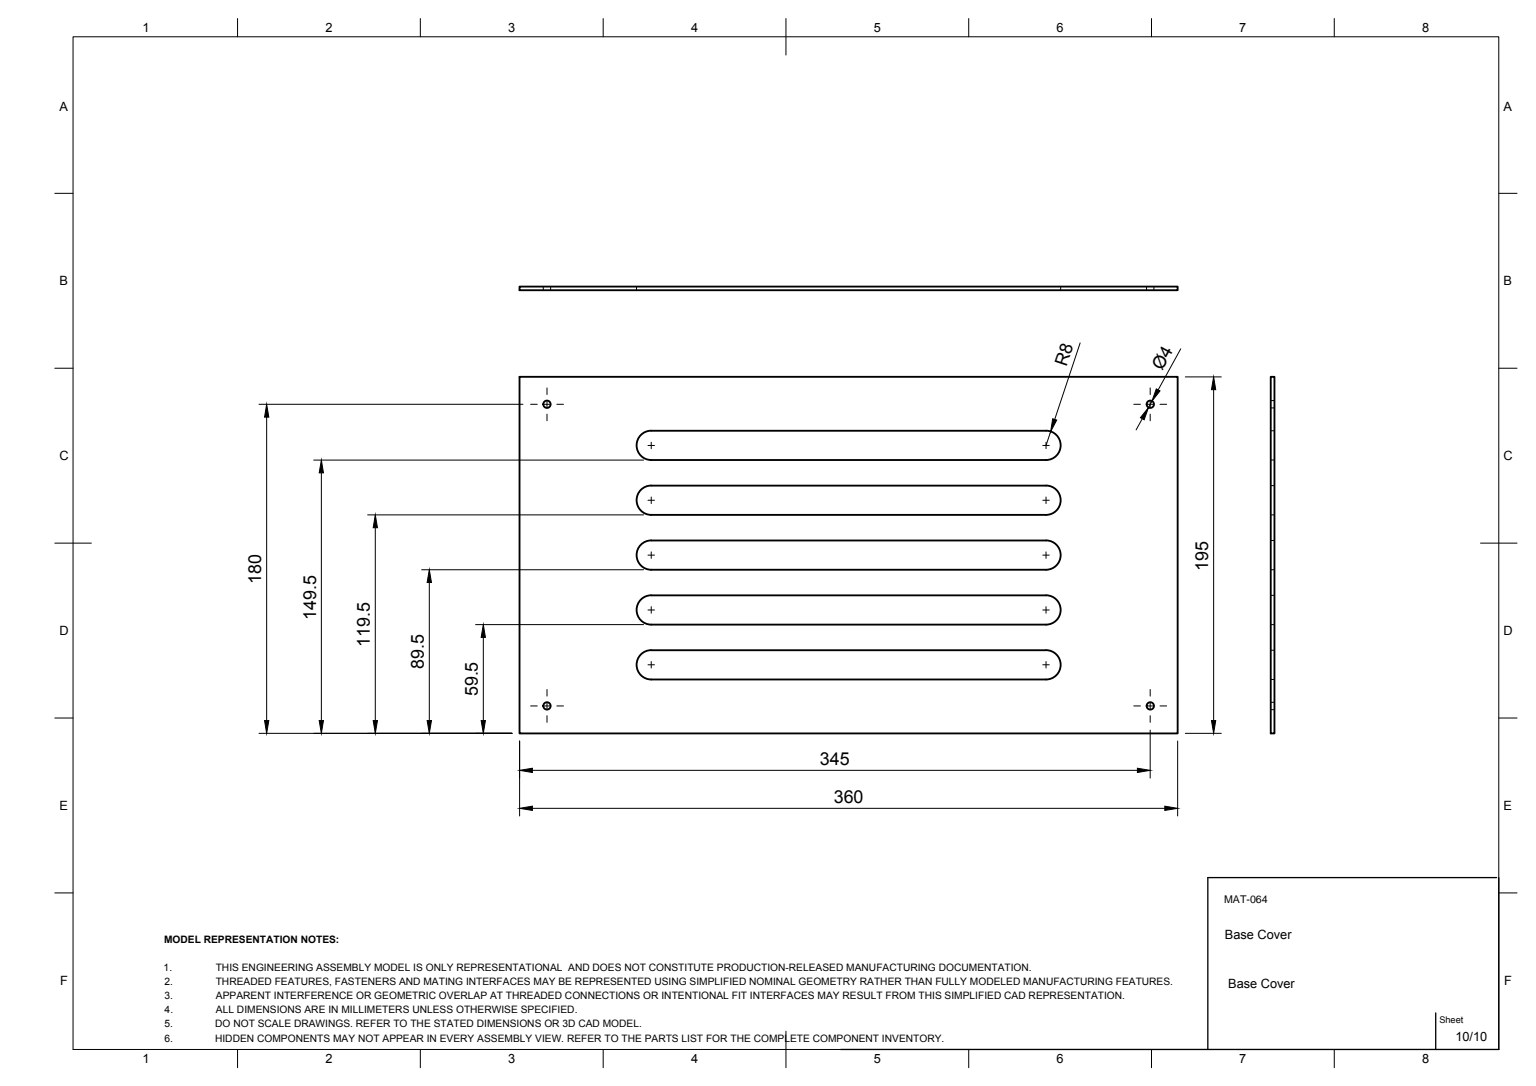
ISO-10303-21;
HEADER;
/* Generated by software containing ST-Developer
 * from STEP Tools, Inc. (www.steptools.com) 
 */

FILE_DESCRIPTION(
/* description */ (''),
/* implementation_level */ '2;1');

FILE_NAME(
/* name */ 
'Base Cover.step',
/* time_stamp */ '2026-10-24T12:42:14-07:00',
/* author */ (''),
/* organization */ (''),
/* preprocessor_version */ 'ST-DEVELOPER v20.2',
/* originating_system */ 'Autodesk Translation Framework v15.15.0.0',
/* authorisation */ '');

FILE_SCHEMA (('AUTOMOTIVE_DESIGN { 1 0 10303 214 3 1 1 }'));
ENDSEC;

DATA;
#10=MECHANICAL_DESIGN_GEOMETRIC_PRESENTATION_REPRESENTATION('',(#67),#6789);
#55=SHAPE_REPRESENTATION_RELATIONSHIP('SRR','None',#6822,#61);
#61=ADVANCED_BREP_SHAPE_REPRESENTATION('',(#73),#6784);
#67=STYLED_ITEM('',(#6863),#73);
#73=MANIFOLD_SOLID_BREP('Base Cover',#3962);
#146=CYLINDRICAL_SURFACE('',#4260,2.);
#147=CYLINDRICAL_SURFACE('',#4261,2.);
#148=CYLINDRICAL_SURFACE('',#4262,2.);
#149=CYLINDRICAL_SURFACE('',#4263,2.);
#150=CYLINDRICAL_SURFACE('',#4264,7.99999999999998);
#151=CYLINDRICAL_SURFACE('',#4266,8.00000000000009);
#152=CYLINDRICAL_SURFACE('',#4268,8.00000000000009);
#153=CYLINDRICAL_SURFACE('',#4270,8.00000000000004);
#154=CYLINDRICAL_SURFACE('',#4272,7.99999999999998);
#155=CYLINDRICAL_SURFACE('',#4274,8.00000000000009);
#156=CYLINDRICAL_SURFACE('',#4276,8.00000000000009);
#157=CYLINDRICAL_SURFACE('',#4278,8.00000000000004);
#158=CYLINDRICAL_SURFACE('',#4280,8.00000000000004);
#159=CYLINDRICAL_SURFACE('',#4282,8.00000000000004);
#201=FACE_BOUND('',#752,.T.);
#202=FACE_BOUND('',#753,.T.);
#203=FACE_BOUND('',#754,.T.);
#204=FACE_BOUND('',#755,.T.);
#205=FACE_BOUND('',#756,.T.);
#206=FACE_BOUND('',#757,.T.);
#207=FACE_BOUND('',#758,.T.);
#208=FACE_BOUND('',#759,.T.);
#209=FACE_BOUND('',#760,.T.);
#210=FACE_BOUND('',#762,.T.);
#211=FACE_BOUND('',#763,.T.);
#212=FACE_BOUND('',#764,.T.);
#213=FACE_BOUND('',#765,.T.);
#214=FACE_BOUND('',#766,.T.);
#215=FACE_BOUND('',#767,.T.);
#216=FACE_BOUND('',#768,.T.);
#217=FACE_BOUND('',#769,.T.);
#218=FACE_BOUND('',#770,.T.);
#294=CIRCLE('',#4231,8.00000000000004);
#295=CIRCLE('',#4232,8.00000000000004);
#296=CIRCLE('',#4233,8.00000000000009);
#297=CIRCLE('',#4234,8.00000000000004);
#298=CIRCLE('',#4235,7.99999999999998);
#299=CIRCLE('',#4236,8.00000000000009);
#300=CIRCLE('',#4237,8.00000000000009);
#301=CIRCLE('',#4238,8.00000000000004);
#302=CIRCLE('',#4239,7.99999999999998);
#303=CIRCLE('',#4240,8.00000000000009);
#304=CIRCLE('',#4241,2.);
#305=CIRCLE('',#4242,2.);
#306=CIRCLE('',#4243,2.);
#307=CIRCLE('',#4244,2.);
#308=CIRCLE('',#4246,8.00000000000004);
#309=CIRCLE('',#4247,8.00000000000004);
#310=CIRCLE('',#4248,8.00000000000009);
#311=CIRCLE('',#4249,8.00000000000004);
#312=CIRCLE('',#4250,7.99999999999998);
#313=CIRCLE('',#4251,8.00000000000009);
#314=CIRCLE('',#4252,8.00000000000009);
#315=CIRCLE('',#4253,8.00000000000004);
#316=CIRCLE('',#4254,7.99999999999998);
#317=CIRCLE('',#4255,8.00000000000009);
#318=CIRCLE('',#4256,2.);
#319=CIRCLE('',#4257,2.);
#320=CIRCLE('',#4258,2.);
#321=CIRCLE('',#4259,2.);
#514=FACE_OUTER_BOUND('',#747,.T.);
#515=FACE_OUTER_BOUND('',#748,.T.);
#516=FACE_OUTER_BOUND('',#749,.T.);
#517=FACE_OUTER_BOUND('',#750,.T.);
#518=FACE_OUTER_BOUND('',#751,.T.);
#519=FACE_OUTER_BOUND('',#761,.T.);
#520=FACE_OUTER_BOUND('',#771,.T.);
#521=FACE_OUTER_BOUND('',#772,.T.);
#522=FACE_OUTER_BOUND('',#773,.T.);
#523=FACE_OUTER_BOUND('',#774,.T.);
#524=FACE_OUTER_BOUND('',#775,.T.);
#525=FACE_OUTER_BOUND('',#776,.T.);
#526=FACE_OUTER_BOUND('',#777,.T.);
#527=FACE_OUTER_BOUND('',#778,.T.);
#528=FACE_OUTER_BOUND('',#779,.T.);
#529=FACE_OUTER_BOUND('',#780,.T.);
#530=FACE_OUTER_BOUND('',#781,.T.);
#531=FACE_OUTER_BOUND('',#782,.T.);
#532=FACE_OUTER_BOUND('',#783,.T.);
#533=FACE_OUTER_BOUND('',#784,.T.);
#534=FACE_OUTER_BOUND('',#785,.T.);
#535=FACE_OUTER_BOUND('',#786,.T.);
#536=FACE_OUTER_BOUND('',#787,.T.);
#537=FACE_OUTER_BOUND('',#788,.T.);
#538=FACE_OUTER_BOUND('',#789,.T.);
#539=FACE_OUTER_BOUND('',#790,.T.);
#540=FACE_OUTER_BOUND('',#791,.T.);
#541=FACE_OUTER_BOUND('',#792,.T.);
#542=FACE_OUTER_BOUND('',#793,.T.);
#543=FACE_OUTER_BOUND('',#794,.T.);
#747=EDGE_LOOP('',(#3177,#3178,#3179,#3180));
#748=EDGE_LOOP('',(#3181,#3182,#3183,#3184));
#749=EDGE_LOOP('',(#3185,#3186,#3187,#3188));
#750=EDGE_LOOP('',(#3189,#3190,#3191,#3192));
#751=EDGE_LOOP('',(#3193,#3194,#3195,#3196));
#752=EDGE_LOOP('',(#3197,#3198,#3199,#3200));
#753=EDGE_LOOP('',(#3201,#3202,#3203,#3204));
#754=EDGE_LOOP('',(#3205,#3206,#3207,#3208));
#755=EDGE_LOOP('',(#3209,#3210,#3211,#3212));
#756=EDGE_LOOP('',(#3213,#3214,#3215,#3216));
#757=EDGE_LOOP('',(#3217));
#758=EDGE_LOOP('',(#3218));
#759=EDGE_LOOP('',(#3219));
#760=EDGE_LOOP('',(#3220));
#761=EDGE_LOOP('',(#3221,#3222,#3223,#3224));
#762=EDGE_LOOP('',(#3225,#3226,#3227,#3228));
#763=EDGE_LOOP('',(#3229,#3230,#3231,#3232));
#764=EDGE_LOOP('',(#3233,#3234,#3235,#3236));
#765=EDGE_LOOP('',(#3237,#3238,#3239,#3240));
#766=EDGE_LOOP('',(#3241,#3242,#3243,#3244));
#767=EDGE_LOOP('',(#3245));
#768=EDGE_LOOP('',(#3246));
#769=EDGE_LOOP('',(#3247));
#770=EDGE_LOOP('',(#3248));
#771=EDGE_LOOP('',(#3249,#3250,#3251,#3252));
#772=EDGE_LOOP('',(#3253,#3254,#3255,#3256));
#773=EDGE_LOOP('',(#3257,#3258,#3259,#3260));
#774=EDGE_LOOP('',(#3261,#3262,#3263,#3264));
#775=EDGE_LOOP('',(#3265,#3266,#3267,#3268));
#776=EDGE_LOOP('',(#3269,#3270,#3271,#3272));
#777=EDGE_LOOP('',(#3273,#3274,#3275,#3276));
#778=EDGE_LOOP('',(#3277,#3278,#3279,#3280));
#779=EDGE_LOOP('',(#3281,#3282,#3283,#3284));
#780=EDGE_LOOP('',(#3285,#3286,#3287,#3288));
#781=EDGE_LOOP('',(#3289,#3290,#3291,#3292));
#782=EDGE_LOOP('',(#3293,#3294,#3295,#3296));
#783=EDGE_LOOP('',(#3297,#3298,#3299,#3300));
#784=EDGE_LOOP('',(#3301,#3302,#3303,#3304));
#785=EDGE_LOOP('',(#3305,#3306,#3307,#3308));
#786=EDGE_LOOP('',(#3309,#3310,#3311,#3312));
#787=EDGE_LOOP('',(#3313,#3314,#3315,#3316));
#788=EDGE_LOOP('',(#3317,#3318,#3319,#3320));
#789=EDGE_LOOP('',(#3321,#3322,#3323,#3324));
#790=EDGE_LOOP('',(#3325,#3326,#3327,#3328));
#791=EDGE_LOOP('',(#3329,#3330,#3331,#3332));
#792=EDGE_LOOP('',(#3333,#3334,#3335,#3336));
#793=EDGE_LOOP('',(#3337,#3338,#3339,#3340));
#794=EDGE_LOOP('',(#3341,#3342,#3343,#3344));
#1139=LINE('',#6259,#1517);
#1140=LINE('',#6261,#1518);
#1141=LINE('',#6263,#1519);
#1142=LINE('',#6264,#1520);
#1143=LINE('',#6267,#1521);
#1144=LINE('',#6269,#1522);
#1145=LINE('',#6270,#1523);
#1146=LINE('',#6273,#1524);
#1147=LINE('',#6275,#1525);
#1148=LINE('',#6276,#1526);
#1149=LINE('',#6278,#1527);
#1150=LINE('',#6279,#1528);
#1151=LINE('',#6285,#1529);
#1152=LINE('',#6288,#1530);
#1153=LINE('',#6293,#1531);
#1154=LINE('',#6296,#1532);
#1155=LINE('',#6301,#1533);
#1156=LINE('',#6304,#1534);
#1157=LINE('',#6309,#1535);
#1158=LINE('',#6312,#1536);
#1159=LINE('',#6317,#1537);
#1160=LINE('',#6320,#1538);
#1161=LINE('',#6332,#1539);
#1162=LINE('',#6336,#1540);
#1163=LINE('',#6340,#1541);
#1164=LINE('',#6344,#1542);
#1165=LINE('',#6348,#1543);
#1166=LINE('',#6352,#1544);
#1167=LINE('',#6356,#1545);
#1168=LINE('',#6360,#1546);
#1169=LINE('',#6364,#1547);
#1170=LINE('',#6368,#1548);
#1171=LINE('',#6379,#1549);
#1172=LINE('',#6381,#1550);
#1173=LINE('',#6383,#1551);
#1174=LINE('',#6385,#1552);
#1175=LINE('',#6387,#1553);
#1176=LINE('',#6388,#1554);
#1177=LINE('',#6390,#1555);
#1178=LINE('',#6392,#1556);
#1179=LINE('',#6395,#1557);
#1180=LINE('',#6396,#1558);
#1181=LINE('',#6398,#1559);
#1182=LINE('',#6400,#1560);
#1183=LINE('',#6403,#1561);
#1184=LINE('',#6404,#1562);
#1185=LINE('',#6406,#1563);
#1186=LINE('',#6408,#1564);
#1187=LINE('',#6411,#1565);
#1188=LINE('',#6412,#1566);
#1189=LINE('',#6414,#1567);
#1190=LINE('',#6416,#1568);
#1191=LINE('',#6419,#1569);
#1192=LINE('',#6420,#1570);
#1193=LINE('',#6422,#1571);
#1194=LINE('',#6424,#1572);
#1517=VECTOR('',#5072,195.);
#1518=VECTOR('',#5073,1.99999999999999);
#1519=VECTOR('',#5074,195.);
#1520=VECTOR('',#5075,1.99999999999999);
#1521=VECTOR('',#5078,360.);
#1522=VECTOR('',#5079,1.99999999999999);
#1523=VECTOR('',#5080,360.);
#1524=VECTOR('',#5083,195.);
#1525=VECTOR('',#5084,1.99999999999999);
#1526=VECTOR('',#5085,195.);
#1527=VECTOR('',#5088,360.);
#1528=VECTOR('',#5089,360.);
#1529=VECTOR('',#5094,216.);
#1530=VECTOR('',#5097,216.);
#1531=VECTOR('',#5100,216.);
#1532=VECTOR('',#5103,216.);
#1533=VECTOR('',#5106,216.);
#1534=VECTOR('',#5109,216.);
#1535=VECTOR('',#5112,216.);
#1536=VECTOR('',#5115,216.);
#1537=VECTOR('',#5118,216.);
#1538=VECTOR('',#5121,216.);
#1539=VECTOR('',#5132,216.);
#1540=VECTOR('',#5135,216.);
#1541=VECTOR('',#5138,216.);
#1542=VECTOR('',#5141,216.);
#1543=VECTOR('',#5144,216.);
#1544=VECTOR('',#5147,216.);
#1545=VECTOR('',#5150,216.);
#1546=VECTOR('',#5153,216.);
#1547=VECTOR('',#5156,216.);
#1548=VECTOR('',#5159,216.);
#1549=VECTOR('',#5172,2.);
#1550=VECTOR('',#5175,2.);
#1551=VECTOR('',#5178,2.);
#1552=VECTOR('',#5181,2.);
#1553=VECTOR('',#5184,1.99999999999999);
#1554=VECTOR('',#5185,1.99999999999999);
#1555=VECTOR('',#5188,1.99999999999999);
#1556=VECTOR('',#5191,1.99999999999999);
#1557=VECTOR('',#5196,1.99999999999999);
#1558=VECTOR('',#5197,1.99999999999999);
#1559=VECTOR('',#5200,1.99999999999999);
#1560=VECTOR('',#5203,1.99999999999999);
#1561=VECTOR('',#5208,1.99999999999999);
#1562=VECTOR('',#5209,1.99999999999999);
#1563=VECTOR('',#5212,1.99999999999999);
#1564=VECTOR('',#5215,1.99999999999999);
#1565=VECTOR('',#5220,1.99999999999999);
#1566=VECTOR('',#5221,1.99999999999999);
#1567=VECTOR('',#5224,1.99999999999999);
#1568=VECTOR('',#5227,1.99999999999999);
#1569=VECTOR('',#5232,1.99999999999999);
#1570=VECTOR('',#5233,1.99999999999999);
#1571=VECTOR('',#5236,1.99999999999999);
#1572=VECTOR('',#5239,1.99999999999999);
#1845=VERTEX_POINT('',#6257);
#1846=VERTEX_POINT('',#6258);
#1847=VERTEX_POINT('',#6260);
#1848=VERTEX_POINT('',#6262);
#1849=VERTEX_POINT('',#6266);
#1850=VERTEX_POINT('',#6268);
#1851=VERTEX_POINT('',#6272);
#1852=VERTEX_POINT('',#6274);
#1853=VERTEX_POINT('',#6281);
#1854=VERTEX_POINT('',#6282);
#1855=VERTEX_POINT('',#6284);
#1856=VERTEX_POINT('',#6286);
#1857=VERTEX_POINT('',#6289);
#1858=VERTEX_POINT('',#6290);
#1859=VERTEX_POINT('',#6292);
#1860=VERTEX_POINT('',#6294);
#1861=VERTEX_POINT('',#6297);
#1862=VERTEX_POINT('',#6298);
#1863=VERTEX_POINT('',#6300);
#1864=VERTEX_POINT('',#6302);
#1865=VERTEX_POINT('',#6305);
#1866=VERTEX_POINT('',#6306);
#1867=VERTEX_POINT('',#6308);
#1868=VERTEX_POINT('',#6310);
#1869=VERTEX_POINT('',#6313);
#1870=VERTEX_POINT('',#6314);
#1871=VERTEX_POINT('',#6316);
#1872=VERTEX_POINT('',#6318);
#1873=VERTEX_POINT('',#6321);
#1874=VERTEX_POINT('',#6323);
#1875=VERTEX_POINT('',#6325);
#1876=VERTEX_POINT('',#6327);
#1877=VERTEX_POINT('',#6330);
#1878=VERTEX_POINT('',#6331);
#1879=VERTEX_POINT('',#6333);
#1880=VERTEX_POINT('',#6335);
#1881=VERTEX_POINT('',#6338);
#1882=VERTEX_POINT('',#6339);
#1883=VERTEX_POINT('',#6341);
#1884=VERTEX_POINT('',#6343);
#1885=VERTEX_POINT('',#6346);
#1886=VERTEX_POINT('',#6347);
#1887=VERTEX_POINT('',#6349);
#1888=VERTEX_POINT('',#6351);
#1889=VERTEX_POINT('',#6354);
#1890=VERTEX_POINT('',#6355);
#1891=VERTEX_POINT('',#6357);
#1892=VERTEX_POINT('',#6359);
#1893=VERTEX_POINT('',#6362);
#1894=VERTEX_POINT('',#6363);
#1895=VERTEX_POINT('',#6365);
#1896=VERTEX_POINT('',#6367);
#1897=VERTEX_POINT('',#6370);
#1898=VERTEX_POINT('',#6372);
#1899=VERTEX_POINT('',#6374);
#1900=VERTEX_POINT('',#6376);
#2309=EDGE_CURVE('',#1845,#1846,#1139,.T.);
#2310=EDGE_CURVE('',#1847,#1846,#1140,.T.);
#2311=EDGE_CURVE('',#1848,#1847,#1141,.T.);
#2312=EDGE_CURVE('',#1848,#1845,#1142,.T.);
#2313=EDGE_CURVE('',#1846,#1849,#1143,.T.);
#2314=EDGE_CURVE('',#1850,#1849,#1144,.T.);
#2315=EDGE_CURVE('',#1847,#1850,#1145,.T.);
#2316=EDGE_CURVE('',#1851,#1849,#1146,.T.);
#2317=EDGE_CURVE('',#1852,#1851,#1147,.T.);
#2318=EDGE_CURVE('',#1852,#1850,#1148,.T.);
#2319=EDGE_CURVE('',#1845,#1851,#1149,.T.);
#2320=EDGE_CURVE('',#1848,#1852,#1150,.T.);
#2321=EDGE_CURVE('',#1853,#1854,#294,.T.);
#2322=EDGE_CURVE('',#1855,#1853,#1151,.T.);
#2323=EDGE_CURVE('',#1856,#1855,#295,.T.);
#2324=EDGE_CURVE('',#1854,#1856,#1152,.T.);
#2325=EDGE_CURVE('',#1857,#1858,#296,.T.);
#2326=EDGE_CURVE('',#1859,#1857,#1153,.T.);
#2327=EDGE_CURVE('',#1860,#1859,#297,.T.);
#2328=EDGE_CURVE('',#1858,#1860,#1154,.T.);
#2329=EDGE_CURVE('',#1861,#1862,#298,.T.);
#2330=EDGE_CURVE('',#1863,#1861,#1155,.T.);
#2331=EDGE_CURVE('',#1864,#1863,#299,.T.);
#2332=EDGE_CURVE('',#1862,#1864,#1156,.T.);
#2333=EDGE_CURVE('',#1865,#1866,#300,.T.);
#2334=EDGE_CURVE('',#1867,#1865,#1157,.T.);
#2335=EDGE_CURVE('',#1868,#1867,#301,.T.);
#2336=EDGE_CURVE('',#1866,#1868,#1158,.T.);
#2337=EDGE_CURVE('',#1869,#1870,#302,.T.);
#2338=EDGE_CURVE('',#1871,#1869,#1159,.T.);
#2339=EDGE_CURVE('',#1872,#1871,#303,.T.);
#2340=EDGE_CURVE('',#1870,#1872,#1160,.T.);
#2341=EDGE_CURVE('',#1873,#1873,#304,.T.);
#2342=EDGE_CURVE('',#1874,#1874,#305,.T.);
#2343=EDGE_CURVE('',#1875,#1875,#306,.T.);
#2344=EDGE_CURVE('',#1876,#1876,#307,.T.);
#2345=EDGE_CURVE('',#1877,#1878,#1161,.T.);
#2346=EDGE_CURVE('',#1878,#1879,#308,.T.);
#2347=EDGE_CURVE('',#1879,#1880,#1162,.T.);
#2348=EDGE_CURVE('',#1880,#1877,#309,.T.);
#2349=EDGE_CURVE('',#1881,#1882,#1163,.T.);
#2350=EDGE_CURVE('',#1882,#1883,#310,.T.);
#2351=EDGE_CURVE('',#1883,#1884,#1164,.T.);
#2352=EDGE_CURVE('',#1884,#1881,#311,.T.);
#2353=EDGE_CURVE('',#1885,#1886,#1165,.T.);
#2354=EDGE_CURVE('',#1886,#1887,#312,.T.);
#2355=EDGE_CURVE('',#1887,#1888,#1166,.T.);
#2356=EDGE_CURVE('',#1888,#1885,#313,.T.);
#2357=EDGE_CURVE('',#1889,#1890,#1167,.T.);
#2358=EDGE_CURVE('',#1890,#1891,#314,.T.);
#2359=EDGE_CURVE('',#1891,#1892,#1168,.T.);
#2360=EDGE_CURVE('',#1892,#1889,#315,.T.);
#2361=EDGE_CURVE('',#1893,#1894,#1169,.T.);
#2362=EDGE_CURVE('',#1894,#1895,#316,.T.);
#2363=EDGE_CURVE('',#1895,#1896,#1170,.T.);
#2364=EDGE_CURVE('',#1896,#1893,#317,.T.);
#2365=EDGE_CURVE('',#1897,#1897,#318,.T.);
#2366=EDGE_CURVE('',#1898,#1898,#319,.T.);
#2367=EDGE_CURVE('',#1899,#1899,#320,.T.);
#2368=EDGE_CURVE('',#1900,#1900,#321,.T.);
#2369=EDGE_CURVE('',#1900,#1876,#1171,.T.);
#2370=EDGE_CURVE('',#1899,#1875,#1172,.T.);
#2371=EDGE_CURVE('',#1898,#1874,#1173,.T.);
#2372=EDGE_CURVE('',#1897,#1873,#1174,.T.);
#2373=EDGE_CURVE('',#1894,#1869,#1175,.T.);
#2374=EDGE_CURVE('',#1895,#1870,#1176,.T.);
#2375=EDGE_CURVE('',#1893,#1871,#1177,.T.);
#2376=EDGE_CURVE('',#1896,#1872,#1178,.T.);
#2377=EDGE_CURVE('',#1890,#1865,#1179,.T.);
#2378=EDGE_CURVE('',#1891,#1866,#1180,.T.);
#2379=EDGE_CURVE('',#1889,#1867,#1181,.T.);
#2380=EDGE_CURVE('',#1892,#1868,#1182,.T.);
#2381=EDGE_CURVE('',#1886,#1861,#1183,.T.);
#2382=EDGE_CURVE('',#1887,#1862,#1184,.T.);
#2383=EDGE_CURVE('',#1885,#1863,#1185,.T.);
#2384=EDGE_CURVE('',#1888,#1864,#1186,.T.);
#2385=EDGE_CURVE('',#1882,#1857,#1187,.T.);
#2386=EDGE_CURVE('',#1883,#1858,#1188,.T.);
#2387=EDGE_CURVE('',#1881,#1859,#1189,.T.);
#2388=EDGE_CURVE('',#1884,#1860,#1190,.T.);
#2389=EDGE_CURVE('',#1878,#1853,#1191,.T.);
#2390=EDGE_CURVE('',#1879,#1854,#1192,.T.);
#2391=EDGE_CURVE('',#1877,#1855,#1193,.T.);
#2392=EDGE_CURVE('',#1880,#1856,#1194,.T.);
#3177=ORIENTED_EDGE('',*,*,#2309,.T.);
#3178=ORIENTED_EDGE('',*,*,#2310,.F.);
#3179=ORIENTED_EDGE('',*,*,#2311,.F.);
#3180=ORIENTED_EDGE('',*,*,#2312,.T.);
#3181=ORIENTED_EDGE('',*,*,#2313,.T.);
#3182=ORIENTED_EDGE('',*,*,#2314,.F.);
#3183=ORIENTED_EDGE('',*,*,#2315,.F.);
#3184=ORIENTED_EDGE('',*,*,#2310,.T.);
#3185=ORIENTED_EDGE('',*,*,#2316,.F.);
#3186=ORIENTED_EDGE('',*,*,#2317,.F.);
#3187=ORIENTED_EDGE('',*,*,#2318,.T.);
#3188=ORIENTED_EDGE('',*,*,#2314,.T.);
#3189=ORIENTED_EDGE('',*,*,#2319,.F.);
#3190=ORIENTED_EDGE('',*,*,#2312,.F.);
#3191=ORIENTED_EDGE('',*,*,#2320,.T.);
#3192=ORIENTED_EDGE('',*,*,#2317,.T.);
#3193=ORIENTED_EDGE('',*,*,#2311,.T.);
#3194=ORIENTED_EDGE('',*,*,#2315,.T.);
#3195=ORIENTED_EDGE('',*,*,#2318,.F.);
#3196=ORIENTED_EDGE('',*,*,#2320,.F.);
#3197=ORIENTED_EDGE('',*,*,#2321,.F.);
#3198=ORIENTED_EDGE('',*,*,#2322,.F.);
#3199=ORIENTED_EDGE('',*,*,#2323,.F.);
#3200=ORIENTED_EDGE('',*,*,#2324,.F.);
#3201=ORIENTED_EDGE('',*,*,#2325,.F.);
#3202=ORIENTED_EDGE('',*,*,#2326,.F.);
#3203=ORIENTED_EDGE('',*,*,#2327,.F.);
#3204=ORIENTED_EDGE('',*,*,#2328,.F.);
#3205=ORIENTED_EDGE('',*,*,#2329,.F.);
#3206=ORIENTED_EDGE('',*,*,#2330,.F.);
#3207=ORIENTED_EDGE('',*,*,#2331,.F.);
#3208=ORIENTED_EDGE('',*,*,#2332,.F.);
#3209=ORIENTED_EDGE('',*,*,#2333,.F.);
#3210=ORIENTED_EDGE('',*,*,#2334,.F.);
#3211=ORIENTED_EDGE('',*,*,#2335,.F.);
#3212=ORIENTED_EDGE('',*,*,#2336,.F.);
#3213=ORIENTED_EDGE('',*,*,#2337,.F.);
#3214=ORIENTED_EDGE('',*,*,#2338,.F.);
#3215=ORIENTED_EDGE('',*,*,#2339,.F.);
#3216=ORIENTED_EDGE('',*,*,#2340,.F.);
#3217=ORIENTED_EDGE('',*,*,#2341,.F.);
#3218=ORIENTED_EDGE('',*,*,#2342,.F.);
#3219=ORIENTED_EDGE('',*,*,#2343,.F.);
#3220=ORIENTED_EDGE('',*,*,#2344,.F.);
#3221=ORIENTED_EDGE('',*,*,#2309,.F.);
#3222=ORIENTED_EDGE('',*,*,#2319,.T.);
#3223=ORIENTED_EDGE('',*,*,#2316,.T.);
#3224=ORIENTED_EDGE('',*,*,#2313,.F.);
#3225=ORIENTED_EDGE('',*,*,#2345,.T.);
#3226=ORIENTED_EDGE('',*,*,#2346,.T.);
#3227=ORIENTED_EDGE('',*,*,#2347,.T.);
#3228=ORIENTED_EDGE('',*,*,#2348,.T.);
#3229=ORIENTED_EDGE('',*,*,#2349,.T.);
#3230=ORIENTED_EDGE('',*,*,#2350,.T.);
#3231=ORIENTED_EDGE('',*,*,#2351,.T.);
#3232=ORIENTED_EDGE('',*,*,#2352,.T.);
#3233=ORIENTED_EDGE('',*,*,#2353,.T.);
#3234=ORIENTED_EDGE('',*,*,#2354,.T.);
#3235=ORIENTED_EDGE('',*,*,#2355,.T.);
#3236=ORIENTED_EDGE('',*,*,#2356,.T.);
#3237=ORIENTED_EDGE('',*,*,#2357,.T.);
#3238=ORIENTED_EDGE('',*,*,#2358,.T.);
#3239=ORIENTED_EDGE('',*,*,#2359,.T.);
#3240=ORIENTED_EDGE('',*,*,#2360,.T.);
#3241=ORIENTED_EDGE('',*,*,#2361,.T.);
#3242=ORIENTED_EDGE('',*,*,#2362,.T.);
#3243=ORIENTED_EDGE('',*,*,#2363,.T.);
#3244=ORIENTED_EDGE('',*,*,#2364,.T.);
#3245=ORIENTED_EDGE('',*,*,#2365,.T.);
#3246=ORIENTED_EDGE('',*,*,#2366,.T.);
#3247=ORIENTED_EDGE('',*,*,#2367,.T.);
#3248=ORIENTED_EDGE('',*,*,#2368,.T.);
#3249=ORIENTED_EDGE('',*,*,#2368,.F.);
#3250=ORIENTED_EDGE('',*,*,#2369,.T.);
#3251=ORIENTED_EDGE('',*,*,#2344,.T.);
#3252=ORIENTED_EDGE('',*,*,#2369,.F.);
#3253=ORIENTED_EDGE('',*,*,#2367,.F.);
#3254=ORIENTED_EDGE('',*,*,#2370,.T.);
#3255=ORIENTED_EDGE('',*,*,#2343,.T.);
#3256=ORIENTED_EDGE('',*,*,#2370,.F.);
#3257=ORIENTED_EDGE('',*,*,#2366,.F.);
#3258=ORIENTED_EDGE('',*,*,#2371,.T.);
#3259=ORIENTED_EDGE('',*,*,#2342,.T.);
#3260=ORIENTED_EDGE('',*,*,#2371,.F.);
#3261=ORIENTED_EDGE('',*,*,#2365,.F.);
#3262=ORIENTED_EDGE('',*,*,#2372,.T.);
#3263=ORIENTED_EDGE('',*,*,#2341,.T.);
#3264=ORIENTED_EDGE('',*,*,#2372,.F.);
#3265=ORIENTED_EDGE('',*,*,#2373,.T.);
#3266=ORIENTED_EDGE('',*,*,#2337,.T.);
#3267=ORIENTED_EDGE('',*,*,#2374,.F.);
#3268=ORIENTED_EDGE('',*,*,#2362,.F.);
#3269=ORIENTED_EDGE('',*,*,#2375,.T.);
#3270=ORIENTED_EDGE('',*,*,#2338,.T.);
#3271=ORIENTED_EDGE('',*,*,#2373,.F.);
#3272=ORIENTED_EDGE('',*,*,#2361,.F.);
#3273=ORIENTED_EDGE('',*,*,#2376,.T.);
#3274=ORIENTED_EDGE('',*,*,#2339,.T.);
#3275=ORIENTED_EDGE('',*,*,#2375,.F.);
#3276=ORIENTED_EDGE('',*,*,#2364,.F.);
#3277=ORIENTED_EDGE('',*,*,#2374,.T.);
#3278=ORIENTED_EDGE('',*,*,#2340,.T.);
#3279=ORIENTED_EDGE('',*,*,#2376,.F.);
#3280=ORIENTED_EDGE('',*,*,#2363,.F.);
#3281=ORIENTED_EDGE('',*,*,#2377,.T.);
#3282=ORIENTED_EDGE('',*,*,#2333,.T.);
#3283=ORIENTED_EDGE('',*,*,#2378,.F.);
#3284=ORIENTED_EDGE('',*,*,#2358,.F.);
#3285=ORIENTED_EDGE('',*,*,#2379,.T.);
#3286=ORIENTED_EDGE('',*,*,#2334,.T.);
#3287=ORIENTED_EDGE('',*,*,#2377,.F.);
#3288=ORIENTED_EDGE('',*,*,#2357,.F.);
#3289=ORIENTED_EDGE('',*,*,#2380,.T.);
#3290=ORIENTED_EDGE('',*,*,#2335,.T.);
#3291=ORIENTED_EDGE('',*,*,#2379,.F.);
#3292=ORIENTED_EDGE('',*,*,#2360,.F.);
#3293=ORIENTED_EDGE('',*,*,#2378,.T.);
#3294=ORIENTED_EDGE('',*,*,#2336,.T.);
#3295=ORIENTED_EDGE('',*,*,#2380,.F.);
#3296=ORIENTED_EDGE('',*,*,#2359,.F.);
#3297=ORIENTED_EDGE('',*,*,#2381,.T.);
#3298=ORIENTED_EDGE('',*,*,#2329,.T.);
#3299=ORIENTED_EDGE('',*,*,#2382,.F.);
#3300=ORIENTED_EDGE('',*,*,#2354,.F.);
#3301=ORIENTED_EDGE('',*,*,#2383,.T.);
#3302=ORIENTED_EDGE('',*,*,#2330,.T.);
#3303=ORIENTED_EDGE('',*,*,#2381,.F.);
#3304=ORIENTED_EDGE('',*,*,#2353,.F.);
#3305=ORIENTED_EDGE('',*,*,#2384,.T.);
#3306=ORIENTED_EDGE('',*,*,#2331,.T.);
#3307=ORIENTED_EDGE('',*,*,#2383,.F.);
#3308=ORIENTED_EDGE('',*,*,#2356,.F.);
#3309=ORIENTED_EDGE('',*,*,#2382,.T.);
#3310=ORIENTED_EDGE('',*,*,#2332,.T.);
#3311=ORIENTED_EDGE('',*,*,#2384,.F.);
#3312=ORIENTED_EDGE('',*,*,#2355,.F.);
#3313=ORIENTED_EDGE('',*,*,#2385,.T.);
#3314=ORIENTED_EDGE('',*,*,#2325,.T.);
#3315=ORIENTED_EDGE('',*,*,#2386,.F.);
#3316=ORIENTED_EDGE('',*,*,#2350,.F.);
#3317=ORIENTED_EDGE('',*,*,#2387,.T.);
#3318=ORIENTED_EDGE('',*,*,#2326,.T.);
#3319=ORIENTED_EDGE('',*,*,#2385,.F.);
#3320=ORIENTED_EDGE('',*,*,#2349,.F.);
#3321=ORIENTED_EDGE('',*,*,#2388,.T.);
#3322=ORIENTED_EDGE('',*,*,#2327,.T.);
#3323=ORIENTED_EDGE('',*,*,#2387,.F.);
#3324=ORIENTED_EDGE('',*,*,#2352,.F.);
#3325=ORIENTED_EDGE('',*,*,#2386,.T.);
#3326=ORIENTED_EDGE('',*,*,#2328,.T.);
#3327=ORIENTED_EDGE('',*,*,#2388,.F.);
#3328=ORIENTED_EDGE('',*,*,#2351,.F.);
#3329=ORIENTED_EDGE('',*,*,#2389,.T.);
#3330=ORIENTED_EDGE('',*,*,#2321,.T.);
#3331=ORIENTED_EDGE('',*,*,#2390,.F.);
#3332=ORIENTED_EDGE('',*,*,#2346,.F.);
#3333=ORIENTED_EDGE('',*,*,#2391,.T.);
#3334=ORIENTED_EDGE('',*,*,#2322,.T.);
#3335=ORIENTED_EDGE('',*,*,#2389,.F.);
#3336=ORIENTED_EDGE('',*,*,#2345,.F.);
#3337=ORIENTED_EDGE('',*,*,#2392,.T.);
#3338=ORIENTED_EDGE('',*,*,#2323,.T.);
#3339=ORIENTED_EDGE('',*,*,#2391,.F.);
#3340=ORIENTED_EDGE('',*,*,#2348,.F.);
#3341=ORIENTED_EDGE('',*,*,#2390,.T.);
#3342=ORIENTED_EDGE('',*,*,#2324,.T.);
#3343=ORIENTED_EDGE('',*,*,#2392,.F.);
#3344=ORIENTED_EDGE('',*,*,#2347,.F.);
#3699=PLANE('',#4226);
#3700=PLANE('',#4227);
#3701=PLANE('',#4228);
#3702=PLANE('',#4229);
#3703=PLANE('',#4230);
#3704=PLANE('',#4245);
#3705=PLANE('',#4265);
#3706=PLANE('',#4267);
#3707=PLANE('',#4269);
#3708=PLANE('',#4271);
#3709=PLANE('',#4273);
#3710=PLANE('',#4275);
#3711=PLANE('',#4277);
#3712=PLANE('',#4279);
#3713=PLANE('',#4281);
#3714=PLANE('',#4283);
#3864=ADVANCED_FACE('',(#514),#3699,.F.);
#3865=ADVANCED_FACE('',(#515),#3700,.F.);
#3866=ADVANCED_FACE('',(#516),#3701,.T.);
#3867=ADVANCED_FACE('',(#517),#3702,.T.);
#3868=ADVANCED_FACE('',(#518,#201,#202,#203,#204,#205,#206,#207,#208,#209),
#3703,.T.);
#3869=ADVANCED_FACE('',(#519,#210,#211,#212,#213,#214,#215,#216,#217,#218),
#3704,.F.);
#3870=ADVANCED_FACE('',(#520),#146,.F.);
#3871=ADVANCED_FACE('',(#521),#147,.F.);
#3872=ADVANCED_FACE('',(#522),#148,.F.);
#3873=ADVANCED_FACE('',(#523),#149,.F.);
#3874=ADVANCED_FACE('',(#524),#150,.F.);
#3875=ADVANCED_FACE('',(#525),#3705,.F.);
#3876=ADVANCED_FACE('',(#526),#151,.F.);
#3877=ADVANCED_FACE('',(#527),#3706,.F.);
#3878=ADVANCED_FACE('',(#528),#152,.F.);
#3879=ADVANCED_FACE('',(#529),#3707,.F.);
#3880=ADVANCED_FACE('',(#530),#153,.F.);
#3881=ADVANCED_FACE('',(#531),#3708,.F.);
#3882=ADVANCED_FACE('',(#532),#154,.F.);
#3883=ADVANCED_FACE('',(#533),#3709,.F.);
#3884=ADVANCED_FACE('',(#534),#155,.F.);
#3885=ADVANCED_FACE('',(#535),#3710,.F.);
#3886=ADVANCED_FACE('',(#536),#156,.F.);
#3887=ADVANCED_FACE('',(#537),#3711,.F.);
#3888=ADVANCED_FACE('',(#538),#157,.F.);
#3889=ADVANCED_FACE('',(#539),#3712,.F.);
#3890=ADVANCED_FACE('',(#540),#158,.F.);
#3891=ADVANCED_FACE('',(#541),#3713,.F.);
#3892=ADVANCED_FACE('',(#542),#159,.F.);
#3893=ADVANCED_FACE('',(#543),#3714,.F.);
#3962=CLOSED_SHELL('',(#3864,#3865,#3866,#3867,#3868,#3869,#3870,#3871,
#3872,#3873,#3874,#3875,#3876,#3877,#3878,#3879,#3880,#3881,#3882,#3883,
#3884,#3885,#3886,#3887,#3888,#3889,#3890,#3891,#3892,#3893));
#4225=AXIS2_PLACEMENT_3D('',#6255,#5068,#5069);
#4226=AXIS2_PLACEMENT_3D('',#6256,#5070,#5071);
#4227=AXIS2_PLACEMENT_3D('',#6265,#5076,#5077);
#4228=AXIS2_PLACEMENT_3D('',#6271,#5081,#5082);
#4229=AXIS2_PLACEMENT_3D('',#6277,#5086,#5087);
#4230=AXIS2_PLACEMENT_3D('',#6280,#5090,#5091);
#4231=AXIS2_PLACEMENT_3D('',#6283,#5092,#5093);
#4232=AXIS2_PLACEMENT_3D('',#6287,#5095,#5096);
#4233=AXIS2_PLACEMENT_3D('',#6291,#5098,#5099);
#4234=AXIS2_PLACEMENT_3D('',#6295,#5101,#5102);
#4235=AXIS2_PLACEMENT_3D('',#6299,#5104,#5105);
#4236=AXIS2_PLACEMENT_3D('',#6303,#5107,#5108);
#4237=AXIS2_PLACEMENT_3D('',#6307,#5110,#5111);
#4238=AXIS2_PLACEMENT_3D('',#6311,#5113,#5114);
#4239=AXIS2_PLACEMENT_3D('',#6315,#5116,#5117);
#4240=AXIS2_PLACEMENT_3D('',#6319,#5119,#5120);
#4241=AXIS2_PLACEMENT_3D('',#6322,#5122,#5123);
#4242=AXIS2_PLACEMENT_3D('',#6324,#5124,#5125);
#4243=AXIS2_PLACEMENT_3D('',#6326,#5126,#5127);
#4244=AXIS2_PLACEMENT_3D('',#6328,#5128,#5129);
#4245=AXIS2_PLACEMENT_3D('',#6329,#5130,#5131);
#4246=AXIS2_PLACEMENT_3D('',#6334,#5133,#5134);
#4247=AXIS2_PLACEMENT_3D('',#6337,#5136,#5137);
#4248=AXIS2_PLACEMENT_3D('',#6342,#5139,#5140);
#4249=AXIS2_PLACEMENT_3D('',#6345,#5142,#5143);
#4250=AXIS2_PLACEMENT_3D('',#6350,#5145,#5146);
#4251=AXIS2_PLACEMENT_3D('',#6353,#5148,#5149);
#4252=AXIS2_PLACEMENT_3D('',#6358,#5151,#5152);
#4253=AXIS2_PLACEMENT_3D('',#6361,#5154,#5155);
#4254=AXIS2_PLACEMENT_3D('',#6366,#5157,#5158);
#4255=AXIS2_PLACEMENT_3D('',#6369,#5160,#5161);
#4256=AXIS2_PLACEMENT_3D('',#6371,#5162,#5163);
#4257=AXIS2_PLACEMENT_3D('',#6373,#5164,#5165);
#4258=AXIS2_PLACEMENT_3D('',#6375,#5166,#5167);
#4259=AXIS2_PLACEMENT_3D('',#6377,#5168,#5169);
#4260=AXIS2_PLACEMENT_3D('',#6378,#5170,#5171);
#4261=AXIS2_PLACEMENT_3D('',#6380,#5173,#5174);
#4262=AXIS2_PLACEMENT_3D('',#6382,#5176,#5177);
#4263=AXIS2_PLACEMENT_3D('',#6384,#5179,#5180);
#4264=AXIS2_PLACEMENT_3D('',#6386,#5182,#5183);
#4265=AXIS2_PLACEMENT_3D('',#6389,#5186,#5187);
#4266=AXIS2_PLACEMENT_3D('',#6391,#5189,#5190);
#4267=AXIS2_PLACEMENT_3D('',#6393,#5192,#5193);
#4268=AXIS2_PLACEMENT_3D('',#6394,#5194,#5195);
#4269=AXIS2_PLACEMENT_3D('',#6397,#5198,#5199);
#4270=AXIS2_PLACEMENT_3D('',#6399,#5201,#5202);
#4271=AXIS2_PLACEMENT_3D('',#6401,#5204,#5205);
#4272=AXIS2_PLACEMENT_3D('',#6402,#5206,#5207);
#4273=AXIS2_PLACEMENT_3D('',#6405,#5210,#5211);
#4274=AXIS2_PLACEMENT_3D('',#6407,#5213,#5214);
#4275=AXIS2_PLACEMENT_3D('',#6409,#5216,#5217);
#4276=AXIS2_PLACEMENT_3D('',#6410,#5218,#5219);
#4277=AXIS2_PLACEMENT_3D('',#6413,#5222,#5223);
#4278=AXIS2_PLACEMENT_3D('',#6415,#5225,#5226);
#4279=AXIS2_PLACEMENT_3D('',#6417,#5228,#5229);
#4280=AXIS2_PLACEMENT_3D('',#6418,#5230,#5231);
#4281=AXIS2_PLACEMENT_3D('',#6421,#5234,#5235);
#4282=AXIS2_PLACEMENT_3D('',#6423,#5237,#5238);
#4283=AXIS2_PLACEMENT_3D('',#6425,#5240,#5241);
#5068=DIRECTION('axis',(0.,0.,1.));
#5069=DIRECTION('refdir',(1.,0.,0.));
#5070=DIRECTION('center_axis',(1.,1.42336285208353E-16,0.));
#5071=DIRECTION('ref_axis',(0.,0.,-1.));
#5072=DIRECTION('',(9.10952225333462E-17,-1.,0.));
#5073=DIRECTION('',(0.,0.,-1.));
#5074=DIRECTION('',(9.10952225333462E-17,-1.,0.));
#5075=DIRECTION('',(0.,0.,-1.));
#5076=DIRECTION('center_axis',(0.,1.,0.));
#5077=DIRECTION('ref_axis',(0.,0.,1.));
#5078=DIRECTION('',(1.,0.,0.));
#5079=DIRECTION('',(0.,0.,-1.));
#5080=DIRECTION('',(1.,0.,0.));
#5081=DIRECTION('center_axis',(1.,2.84672570416707E-16,0.));
#5082=DIRECTION('ref_axis',(0.,0.,-1.));
#5083=DIRECTION('',(3.64380890133385E-16,-1.,0.));
#5084=DIRECTION('',(0.,0.,-1.));
#5085=DIRECTION('',(3.64380890133385E-16,-1.,0.));
#5086=DIRECTION('center_axis',(0.,1.,0.));
#5087=DIRECTION('ref_axis',(0.,0.,1.));
#5088=DIRECTION('',(1.,0.,0.));
#5089=DIRECTION('',(1.,0.,0.));
#5090=DIRECTION('center_axis',(0.,0.,1.));
#5091=DIRECTION('ref_axis',(1.,0.,0.));
#5092=DIRECTION('center_axis',(0.,0.,1.));
#5093=DIRECTION('ref_axis',(1.,0.,0.));
#5094=DIRECTION('',(-1.,0.,0.));
#5095=DIRECTION('center_axis',(0.,0.,1.));
#5096=DIRECTION('ref_axis',(1.,0.,0.));
#5097=DIRECTION('',(1.,3.28954970259306E-16,0.));
#5098=DIRECTION('center_axis',(0.,0.,1.));
#5099=DIRECTION('ref_axis',(1.,0.,0.));
#5100=DIRECTION('',(-1.,0.,0.));
#5101=DIRECTION('center_axis',(0.,0.,1.));
#5102=DIRECTION('ref_axis',(1.,0.,0.));
#5103=DIRECTION('',(1.,3.28954970259306E-16,0.));
#5104=DIRECTION('center_axis',(0.,0.,1.));
#5105=DIRECTION('ref_axis',(1.,0.,0.));
#5106=DIRECTION('',(-1.,-6.57909940518611E-16,0.));
#5107=DIRECTION('center_axis',(0.,0.,1.));
#5108=DIRECTION('ref_axis',(1.,0.,0.));
#5109=DIRECTION('',(1.,-3.28954970259306E-16,0.));
#5110=DIRECTION('center_axis',(0.,0.,1.));
#5111=DIRECTION('ref_axis',(1.,0.,0.));
#5112=DIRECTION('',(-1.,0.,0.));
#5113=DIRECTION('center_axis',(0.,0.,1.));
#5114=DIRECTION('ref_axis',(1.,0.,0.));
#5115=DIRECTION('',(1.,6.57909940518611E-16,0.));
#5116=DIRECTION('center_axis',(0.,0.,1.));
#5117=DIRECTION('ref_axis',(1.,0.,0.));
#5118=DIRECTION('',(-1.,-6.57909940518611E-16,0.));
#5119=DIRECTION('center_axis',(0.,0.,1.));
#5120=DIRECTION('ref_axis',(1.,0.,0.));
#5121=DIRECTION('',(1.,0.,0.));
#5122=DIRECTION('center_axis',(0.,0.,1.));
#5123=DIRECTION('ref_axis',(1.,0.,0.));
#5124=DIRECTION('center_axis',(0.,0.,1.));
#5125=DIRECTION('ref_axis',(-1.,0.,0.));
#5126=DIRECTION('center_axis',(0.,0.,1.));
#5127=DIRECTION('ref_axis',(-1.,0.,0.));
#5128=DIRECTION('center_axis',(0.,0.,1.));
#5129=DIRECTION('ref_axis',(1.,0.,0.));
#5130=DIRECTION('center_axis',(0.,0.,1.));
#5131=DIRECTION('ref_axis',(1.,0.,0.));
#5132=DIRECTION('',(-1.,0.,0.));
#5133=DIRECTION('center_axis',(0.,0.,1.));
#5134=DIRECTION('ref_axis',(1.,0.,0.));
#5135=DIRECTION('',(1.,3.28954970259306E-16,0.));
#5136=DIRECTION('center_axis',(0.,0.,1.));
#5137=DIRECTION('ref_axis',(1.,0.,0.));
#5138=DIRECTION('',(-1.,0.,0.));
#5139=DIRECTION('center_axis',(0.,0.,1.));
#5140=DIRECTION('ref_axis',(1.,0.,0.));
#5141=DIRECTION('',(1.,3.28954970259306E-16,0.));
#5142=DIRECTION('center_axis',(0.,0.,1.));
#5143=DIRECTION('ref_axis',(1.,0.,0.));
#5144=DIRECTION('',(-1.,-6.57909940518611E-16,0.));
#5145=DIRECTION('center_axis',(0.,0.,1.));
#5146=DIRECTION('ref_axis',(1.,0.,0.));
#5147=DIRECTION('',(1.,-3.28954970259306E-16,0.));
#5148=DIRECTION('center_axis',(0.,0.,1.));
#5149=DIRECTION('ref_axis',(1.,0.,0.));
#5150=DIRECTION('',(-1.,0.,0.));
#5151=DIRECTION('center_axis',(0.,0.,1.));
#5152=DIRECTION('ref_axis',(1.,0.,0.));
#5153=DIRECTION('',(1.,6.57909940518611E-16,0.));
#5154=DIRECTION('center_axis',(0.,0.,1.));
#5155=DIRECTION('ref_axis',(1.,0.,0.));
#5156=DIRECTION('',(-1.,-6.57909940518611E-16,0.));
#5157=DIRECTION('center_axis',(0.,0.,1.));
#5158=DIRECTION('ref_axis',(1.,0.,0.));
#5159=DIRECTION('',(1.,0.,0.));
#5160=DIRECTION('center_axis',(0.,0.,1.));
#5161=DIRECTION('ref_axis',(1.,0.,0.));
#5162=DIRECTION('center_axis',(0.,0.,1.));
#5163=DIRECTION('ref_axis',(1.,0.,0.));
#5164=DIRECTION('center_axis',(0.,0.,1.));
#5165=DIRECTION('ref_axis',(1.,0.,0.));
#5166=DIRECTION('center_axis',(0.,0.,1.));
#5167=DIRECTION('ref_axis',(1.,0.,0.));
#5168=DIRECTION('center_axis',(0.,0.,1.));
#5169=DIRECTION('ref_axis',(1.,0.,0.));
#5170=DIRECTION('center_axis',(0.,0.,1.));
#5171=DIRECTION('ref_axis',(1.,0.,0.));
#5172=DIRECTION('',(0.,0.,1.));
#5173=DIRECTION('center_axis',(0.,0.,1.));
#5174=DIRECTION('ref_axis',(1.,0.,0.));
#5175=DIRECTION('',(0.,0.,1.));
#5176=DIRECTION('center_axis',(0.,0.,1.));
#5177=DIRECTION('ref_axis',(1.,0.,0.));
#5178=DIRECTION('',(0.,0.,1.));
#5179=DIRECTION('center_axis',(0.,0.,1.));
#5180=DIRECTION('ref_axis',(1.,0.,0.));
#5181=DIRECTION('',(0.,0.,1.));
#5182=DIRECTION('center_axis',(0.,0.,1.));
#5183=DIRECTION('ref_axis',(-1.,1.22464679914735E-16,0.));
#5184=DIRECTION('',(0.,0.,1.));
#5185=DIRECTION('',(0.,0.,1.));
#5186=DIRECTION('center_axis',(-7.70988211545248E-16,1.,0.));
#5187=DIRECTION('ref_axis',(0.,0.,1.));
#5188=DIRECTION('',(0.,0.,1.));
#5189=DIRECTION('center_axis',(0.,0.,1.));
#5190=DIRECTION('ref_axis',(1.,0.,0.));
#5191=DIRECTION('',(0.,0.,1.));
#5192=DIRECTION('center_axis',(-2.56996070515083E-16,-1.,0.));
#5193=DIRECTION('ref_axis',(0.,0.,-1.));
#5194=DIRECTION('center_axis',(0.,0.,1.));
#5195=DIRECTION('ref_axis',(-1.,1.22464679914735E-16,0.));
#5196=DIRECTION('',(0.,0.,1.));
#5197=DIRECTION('',(0.,0.,1.));
#5198=DIRECTION('center_axis',(0.,1.,0.));
#5199=DIRECTION('ref_axis',(0.,0.,1.));
#5200=DIRECTION('',(0.,0.,1.));
#5201=DIRECTION('center_axis',(0.,0.,1.));
#5202=DIRECTION('ref_axis',(1.,0.,0.));
#5203=DIRECTION('',(0.,0.,1.));
#5204=DIRECTION('center_axis',(5.13992141030165E-16,-1.,0.));
#5205=DIRECTION('ref_axis',(0.,0.,-1.));
#5206=DIRECTION('center_axis',(0.,0.,1.));
#5207=DIRECTION('ref_axis',(-1.,1.22464679914735E-16,0.));
#5208=DIRECTION('',(0.,0.,1.));
#5209=DIRECTION('',(0.,0.,1.));
#5210=DIRECTION('center_axis',(-7.70988211545248E-16,1.,0.));
#5211=DIRECTION('ref_axis',(0.,0.,1.));
#5212=DIRECTION('',(0.,0.,1.));
#5213=DIRECTION('center_axis',(0.,0.,1.));
#5214=DIRECTION('ref_axis',(1.,0.,0.));
#5215=DIRECTION('',(0.,0.,1.));
#5216=DIRECTION('center_axis',(-2.56996070515083E-16,-1.,0.));
#5217=DIRECTION('ref_axis',(0.,0.,-1.));
#5218=DIRECTION('center_axis',(0.,0.,1.));
#5219=DIRECTION('ref_axis',(-1.,1.22464679914735E-16,0.));
#5220=DIRECTION('',(0.,0.,1.));
#5221=DIRECTION('',(0.,0.,1.));
#5222=DIRECTION('center_axis',(0.,1.,0.));
#5223=DIRECTION('ref_axis',(0.,0.,1.));
#5224=DIRECTION('',(0.,0.,1.));
#5225=DIRECTION('center_axis',(0.,0.,1.));
#5226=DIRECTION('ref_axis',(1.,0.,0.));
#5227=DIRECTION('',(0.,0.,1.));
#5228=DIRECTION('center_axis',(5.13992141030165E-16,-1.,0.));
#5229=DIRECTION('ref_axis',(0.,0.,-1.));
#5230=DIRECTION('center_axis',(0.,0.,1.));
#5231=DIRECTION('ref_axis',(-1.,1.22464679914735E-16,0.));
#5232=DIRECTION('',(0.,0.,1.));
#5233=DIRECTION('',(0.,0.,1.));
#5234=DIRECTION('center_axis',(-2.56996070515083E-16,1.,0.));
#5235=DIRECTION('ref_axis',(0.,0.,1.));
#5236=DIRECTION('',(0.,0.,1.));
#5237=DIRECTION('center_axis',(0.,0.,1.));
#5238=DIRECTION('ref_axis',(1.,0.,0.));
#5239=DIRECTION('',(0.,0.,1.));
#5240=DIRECTION('center_axis',(2.56996070515083E-16,-1.,0.));
#5241=DIRECTION('ref_axis',(0.,0.,-1.));
#6255=CARTESIAN_POINT('',(0.,0.,0.));
#6256=CARTESIAN_POINT('Origin',(-135.,-310.693069306929,302.));
#6257=CARTESIAN_POINT('',(-135.,-310.693069306929,300.));
#6258=CARTESIAN_POINT('',(-135.,-505.693069306929,300.));
#6259=CARTESIAN_POINT('',(-135.,-310.693069306929,300.));
#6260=CARTESIAN_POINT('',(-135.,-505.693069306929,302.));
#6261=CARTESIAN_POINT('',(-135.,-505.693069306929,302.));
#6262=CARTESIAN_POINT('',(-135.,-310.693069306929,302.));
#6263=CARTESIAN_POINT('',(-135.,-310.693069306929,302.));
#6264=CARTESIAN_POINT('',(-135.,-310.693069306929,302.));
#6265=CARTESIAN_POINT('Origin',(-135.,-505.693069306929,302.));
#6266=CARTESIAN_POINT('',(225.,-505.693069306929,300.));
#6267=CARTESIAN_POINT('',(-135.,-505.693069306929,300.));
#6268=CARTESIAN_POINT('',(225.,-505.693069306929,302.));
#6269=CARTESIAN_POINT('',(225.,-505.693069306929,302.));
#6270=CARTESIAN_POINT('',(-135.,-505.693069306929,302.));
#6271=CARTESIAN_POINT('Origin',(225.,-310.693069306929,302.));
#6272=CARTESIAN_POINT('',(225.,-310.693069306929,300.));
#6273=CARTESIAN_POINT('',(225.,-310.693069306929,300.));
#6274=CARTESIAN_POINT('',(225.,-310.693069306929,302.));
#6275=CARTESIAN_POINT('',(225.,-310.693069306929,302.));
#6276=CARTESIAN_POINT('',(225.,-310.693069306929,302.));
#6277=CARTESIAN_POINT('Origin',(-135.,-310.693069306929,302.));
#6278=CARTESIAN_POINT('',(-135.,-310.693069306929,300.));
#6279=CARTESIAN_POINT('',(-135.,-310.693069306929,302.));
#6280=CARTESIAN_POINT('Origin',(0.,0.,302.));
#6281=CARTESIAN_POINT('',(-62.9999999999999,-400.193069306929,302.));
#6282=CARTESIAN_POINT('',(-62.9999999999999,-416.193069306929,302.));
#6283=CARTESIAN_POINT('Origin',(-62.9999999999999,-408.193069306929,302.));
#6284=CARTESIAN_POINT('',(153.,-400.193069306929,302.));
#6285=CARTESIAN_POINT('',(153.,-400.193069306929,302.));
#6286=CARTESIAN_POINT('',(153.,-416.193069306929,302.));
#6287=CARTESIAN_POINT('Origin',(153.,-408.193069306929,302.));
#6288=CARTESIAN_POINT('',(-62.9999999999999,-416.193069306929,302.));
#6289=CARTESIAN_POINT('',(-63.,-370.193069306929,302.));
#6290=CARTESIAN_POINT('',(-63.,-386.193069306929,302.));
#6291=CARTESIAN_POINT('Origin',(-63.,-378.193069306929,302.));
#6292=CARTESIAN_POINT('',(153.,-370.193069306929,302.));
#6293=CARTESIAN_POINT('',(153.,-370.193069306929,302.));
#6294=CARTESIAN_POINT('',(153.,-386.193069306929,302.));
#6295=CARTESIAN_POINT('Origin',(153.,-378.193069306929,302.));
#6296=CARTESIAN_POINT('',(-63.,-386.193069306929,302.));
#6297=CARTESIAN_POINT('',(-63.0000000000001,-340.193069306929,302.));
#6298=CARTESIAN_POINT('',(-63.0000000000001,-356.193069306929,302.));
#6299=CARTESIAN_POINT('Origin',(-63.0000000000001,-348.193069306929,302.));
#6300=CARTESIAN_POINT('',(153.,-340.193069306929,302.));
#6301=CARTESIAN_POINT('',(153.,-340.193069306929,302.));
#6302=CARTESIAN_POINT('',(153.,-356.193069306929,302.));
#6303=CARTESIAN_POINT('Origin',(153.,-348.193069306929,302.));
#6304=CARTESIAN_POINT('',(-63.0000000000001,-356.193069306929,302.));
#6305=CARTESIAN_POINT('',(-62.9999999999996,-430.193069306929,302.));
#6306=CARTESIAN_POINT('',(-62.9999999999996,-446.193069306929,302.));
#6307=CARTESIAN_POINT('Origin',(-62.9999999999996,-438.193069306929,302.));
#6308=CARTESIAN_POINT('',(153.,-430.193069306929,302.));
#6309=CARTESIAN_POINT('',(153.,-430.193069306929,302.));
#6310=CARTESIAN_POINT('',(153.,-446.193069306929,302.));
#6311=CARTESIAN_POINT('Origin',(153.,-438.193069306929,302.));
#6312=CARTESIAN_POINT('',(-62.9999999999996,-446.193069306929,302.));
#6313=CARTESIAN_POINT('',(-62.9999999999993,-460.193069306929,302.));
#6314=CARTESIAN_POINT('',(-62.9999999999993,-476.193069306929,302.));
#6315=CARTESIAN_POINT('Origin',(-62.9999999999993,-468.193069306929,302.));
#6316=CARTESIAN_POINT('',(153.000000000001,-460.193069306928,302.));
#6317=CARTESIAN_POINT('',(153.000000000001,-460.193069306928,302.));
#6318=CARTESIAN_POINT('',(153.000000000001,-476.193069306929,302.));
#6319=CARTESIAN_POINT('Origin',(153.000000000001,-468.193069306929,302.));
#6320=CARTESIAN_POINT('',(-62.9999999999993,-476.193069306929,302.));
#6321=CARTESIAN_POINT('',(208.,-325.693069306929,302.));
#6322=CARTESIAN_POINT('Origin',(210.,-325.693069306929,302.));
#6323=CARTESIAN_POINT('',(-122.,-325.693069306929,302.));
#6324=CARTESIAN_POINT('Origin',(-120.,-325.693069306929,302.));
#6325=CARTESIAN_POINT('',(208.,-490.693069306929,302.));
#6326=CARTESIAN_POINT('Origin',(210.,-490.693069306929,302.));
#6327=CARTESIAN_POINT('',(-122.,-490.693069306929,302.));
#6328=CARTESIAN_POINT('Origin',(-120.,-490.693069306929,302.));
#6329=CARTESIAN_POINT('Origin',(0.,0.,300.));
#6330=CARTESIAN_POINT('',(153.,-400.193069306929,300.));
#6331=CARTESIAN_POINT('',(-62.9999999999999,-400.193069306929,300.));
#6332=CARTESIAN_POINT('',(153.,-400.193069306929,300.));
#6333=CARTESIAN_POINT('',(-62.9999999999999,-416.193069306929,300.));
#6334=CARTESIAN_POINT('Origin',(-62.9999999999999,-408.193069306929,300.));
#6335=CARTESIAN_POINT('',(153.,-416.193069306929,300.));
#6336=CARTESIAN_POINT('',(-62.9999999999999,-416.193069306929,300.));
#6337=CARTESIAN_POINT('Origin',(153.,-408.193069306929,300.));
#6338=CARTESIAN_POINT('',(153.,-370.193069306929,300.));
#6339=CARTESIAN_POINT('',(-63.,-370.193069306929,300.));
#6340=CARTESIAN_POINT('',(153.,-370.193069306929,300.));
#6341=CARTESIAN_POINT('',(-63.,-386.193069306929,300.));
#6342=CARTESIAN_POINT('Origin',(-63.,-378.193069306929,300.));
#6343=CARTESIAN_POINT('',(153.,-386.193069306929,300.));
#6344=CARTESIAN_POINT('',(-63.,-386.193069306929,300.));
#6345=CARTESIAN_POINT('Origin',(153.,-378.193069306929,300.));
#6346=CARTESIAN_POINT('',(153.,-340.193069306929,300.));
#6347=CARTESIAN_POINT('',(-63.0000000000001,-340.193069306929,300.));
#6348=CARTESIAN_POINT('',(153.,-340.193069306929,300.));
#6349=CARTESIAN_POINT('',(-63.0000000000001,-356.193069306929,300.));
#6350=CARTESIAN_POINT('Origin',(-63.0000000000001,-348.193069306929,300.));
#6351=CARTESIAN_POINT('',(153.,-356.193069306929,300.));
#6352=CARTESIAN_POINT('',(-63.0000000000001,-356.193069306929,300.));
#6353=CARTESIAN_POINT('Origin',(153.,-348.193069306929,300.));
#6354=CARTESIAN_POINT('',(153.,-430.193069306929,300.));
#6355=CARTESIAN_POINT('',(-62.9999999999996,-430.193069306929,300.));
#6356=CARTESIAN_POINT('',(153.,-430.193069306929,300.));
#6357=CARTESIAN_POINT('',(-62.9999999999996,-446.193069306929,300.));
#6358=CARTESIAN_POINT('Origin',(-62.9999999999996,-438.193069306929,300.));
#6359=CARTESIAN_POINT('',(153.,-446.193069306929,300.));
#6360=CARTESIAN_POINT('',(-62.9999999999996,-446.193069306929,300.));
#6361=CARTESIAN_POINT('Origin',(153.,-438.193069306929,300.));
#6362=CARTESIAN_POINT('',(153.000000000001,-460.193069306928,300.));
#6363=CARTESIAN_POINT('',(-62.9999999999993,-460.193069306929,300.));
#6364=CARTESIAN_POINT('',(153.000000000001,-460.193069306928,300.));
#6365=CARTESIAN_POINT('',(-62.9999999999993,-476.193069306929,300.));
#6366=CARTESIAN_POINT('Origin',(-62.9999999999993,-468.193069306929,300.));
#6367=CARTESIAN_POINT('',(153.000000000001,-476.193069306929,300.));
#6368=CARTESIAN_POINT('',(-62.9999999999993,-476.193069306929,300.));
#6369=CARTESIAN_POINT('Origin',(153.000000000001,-468.193069306929,300.));
#6370=CARTESIAN_POINT('',(208.,-325.693069306929,300.));
#6371=CARTESIAN_POINT('Origin',(210.,-325.693069306929,300.));
#6372=CARTESIAN_POINT('',(-122.,-325.693069306929,300.));
#6373=CARTESIAN_POINT('Origin',(-120.,-325.693069306929,300.));
#6374=CARTESIAN_POINT('',(208.,-490.693069306929,300.));
#6375=CARTESIAN_POINT('Origin',(210.,-490.693069306929,300.));
#6376=CARTESIAN_POINT('',(-122.,-490.693069306929,300.));
#6377=CARTESIAN_POINT('Origin',(-120.,-490.693069306929,300.));
#6378=CARTESIAN_POINT('Origin',(-120.,-490.693069306929,280.));
#6379=CARTESIAN_POINT('',(-122.,-490.693069306929,280.));
#6380=CARTESIAN_POINT('Origin',(210.,-490.693069306929,280.));
#6381=CARTESIAN_POINT('',(208.,-490.693069306929,280.));
#6382=CARTESIAN_POINT('Origin',(-120.,-325.693069306929,280.));
#6383=CARTESIAN_POINT('',(-122.,-325.693069306929,280.));
#6384=CARTESIAN_POINT('Origin',(210.,-325.693069306929,280.));
#6385=CARTESIAN_POINT('',(208.,-325.693069306929,280.));
#6386=CARTESIAN_POINT('Origin',(-62.9999999999993,-468.193069306929,280.));
#6387=CARTESIAN_POINT('',(-62.9999999999993,-460.193069306929,300.));
#6388=CARTESIAN_POINT('',(-62.9999999999993,-476.193069306929,300.));
#6389=CARTESIAN_POINT('Origin',(-62.9999999999993,-460.193069306929,280.));
#6390=CARTESIAN_POINT('',(153.000000000001,-460.193069306928,300.));
#6391=CARTESIAN_POINT('Origin',(153.000000000001,-468.193069306929,280.));
#6392=CARTESIAN_POINT('',(153.000000000001,-476.193069306929,300.));
#6393=CARTESIAN_POINT('Origin',(-62.9999999999993,-476.193069306929,280.));
#6394=CARTESIAN_POINT('Origin',(-62.9999999999996,-438.193069306929,280.));
#6395=CARTESIAN_POINT('',(-62.9999999999996,-430.193069306929,300.));
#6396=CARTESIAN_POINT('',(-62.9999999999996,-446.193069306929,300.));
#6397=CARTESIAN_POINT('Origin',(-62.9999999999996,-430.193069306929,280.));
#6398=CARTESIAN_POINT('',(153.,-430.193069306929,300.));
#6399=CARTESIAN_POINT('Origin',(153.,-438.193069306929,280.));
#6400=CARTESIAN_POINT('',(153.,-446.193069306929,300.));
#6401=CARTESIAN_POINT('Origin',(-62.9999999999996,-446.193069306929,280.));
#6402=CARTESIAN_POINT('Origin',(-63.0000000000001,-348.193069306929,280.));
#6403=CARTESIAN_POINT('',(-63.0000000000001,-340.193069306929,300.));
#6404=CARTESIAN_POINT('',(-63.0000000000001,-356.193069306929,300.));
#6405=CARTESIAN_POINT('Origin',(-63.0000000000001,-340.193069306929,280.));
#6406=CARTESIAN_POINT('',(153.,-340.193069306929,300.));
#6407=CARTESIAN_POINT('Origin',(153.,-348.193069306929,280.));
#6408=CARTESIAN_POINT('',(153.,-356.193069306929,300.));
#6409=CARTESIAN_POINT('Origin',(-63.0000000000001,-356.193069306929,280.));
#6410=CARTESIAN_POINT('Origin',(-63.,-378.193069306929,280.));
#6411=CARTESIAN_POINT('',(-63.,-370.193069306929,300.));
#6412=CARTESIAN_POINT('',(-63.,-386.193069306929,300.));
#6413=CARTESIAN_POINT('Origin',(-63.,-370.193069306929,280.));
#6414=CARTESIAN_POINT('',(153.,-370.193069306929,300.));
#6415=CARTESIAN_POINT('Origin',(153.,-378.193069306929,280.));
#6416=CARTESIAN_POINT('',(153.,-386.193069306929,300.));
#6417=CARTESIAN_POINT('Origin',(-63.,-386.193069306929,280.));
#6418=CARTESIAN_POINT('Origin',(-62.9999999999999,-408.193069306929,280.));
#6419=CARTESIAN_POINT('',(-62.9999999999999,-400.193069306929,300.));
#6420=CARTESIAN_POINT('',(-62.9999999999999,-416.193069306929,300.));
#6421=CARTESIAN_POINT('Origin',(-62.9999999999999,-400.193069306929,280.));
#6422=CARTESIAN_POINT('',(153.,-400.193069306929,300.));
#6423=CARTESIAN_POINT('Origin',(153.,-408.193069306929,280.));
#6424=CARTESIAN_POINT('',(153.,-416.193069306929,300.));
#6425=CARTESIAN_POINT('Origin',(-62.9999999999999,-416.193069306929,280.));
#6775=UNCERTAINTY_MEASURE_WITH_UNIT(LENGTH_MEASURE(0.01),#6790,
'DISTANCE_ACCURACY_VALUE',
'Maximum model space distance between geometric entities at asserted c
onnectivities');
#6780=UNCERTAINTY_MEASURE_WITH_UNIT(LENGTH_MEASURE(0.01),#6790,
'DISTANCE_ACCURACY_VALUE',
'Maximum model space distance between geometric entities at asserted c
onnectivities');
#6784=(
GEOMETRIC_REPRESENTATION_CONTEXT(3)
GLOBAL_UNCERTAINTY_ASSIGNED_CONTEXT((#6775))
GLOBAL_UNIT_ASSIGNED_CONTEXT((#6790,#6792,#6793))
REPRESENTATION_CONTEXT('','3D')
);
#6789=(
GEOMETRIC_REPRESENTATION_CONTEXT(3)
GLOBAL_UNCERTAINTY_ASSIGNED_CONTEXT((#6780))
GLOBAL_UNIT_ASSIGNED_CONTEXT((#6790,#6792,#6793))
REPRESENTATION_CONTEXT('','3D')
);
#6790=(
LENGTH_UNIT()
NAMED_UNIT(*)
SI_UNIT(.MILLI.,.METRE.)
);
#6792=(
NAMED_UNIT(*)
PLANE_ANGLE_UNIT()
SI_UNIT($,.RADIAN.)
);
#6793=(
NAMED_UNIT(*)
SI_UNIT($,.STERADIAN.)
SOLID_ANGLE_UNIT()
);
#6797=SHAPE_DEFINITION_REPRESENTATION(#6805,#6822);
#6805=PRODUCT_DEFINITION_SHAPE('',$,#6831);
#6822=SHAPE_REPRESENTATION('',(#4225),#6784);
#6827=PRODUCT_DEFINITION_CONTEXT('part definition',#6853,'design');
#6831=PRODUCT_DEFINITION('Base Cover','Base Cover',#6839,#6827);
#6839=PRODUCT_DEFINITION_FORMATION('',$,#6858);
#6853=APPLICATION_CONTEXT(
'Core Data for Automotive Mechanical Design Process');
#6854=PRODUCT_CONTEXT('part definition',#6853,'mechanical');
#6858=PRODUCT('Base Cover','Base Cover',$,(#6854));
#6863=PRESENTATION_STYLE_ASSIGNMENT((#6865));
#6865=SURFACE_STYLE_USAGE(.BOTH.,#6867);
#6867=SURFACE_SIDE_STYLE('',(#6869));
#6869=SURFACE_STYLE_FILL_AREA(#6871);
#6871=FILL_AREA_STYLE('Steel - Satin',(#6873));
#6873=FILL_AREA_STYLE_COLOUR('Steel - Satin',#6875);
#6875=COLOUR_RGB('Steel - Satin',0.627450980392157,0.627450980392157,0.627450980392157);
ENDSEC;
END-ISO-10303-21;
